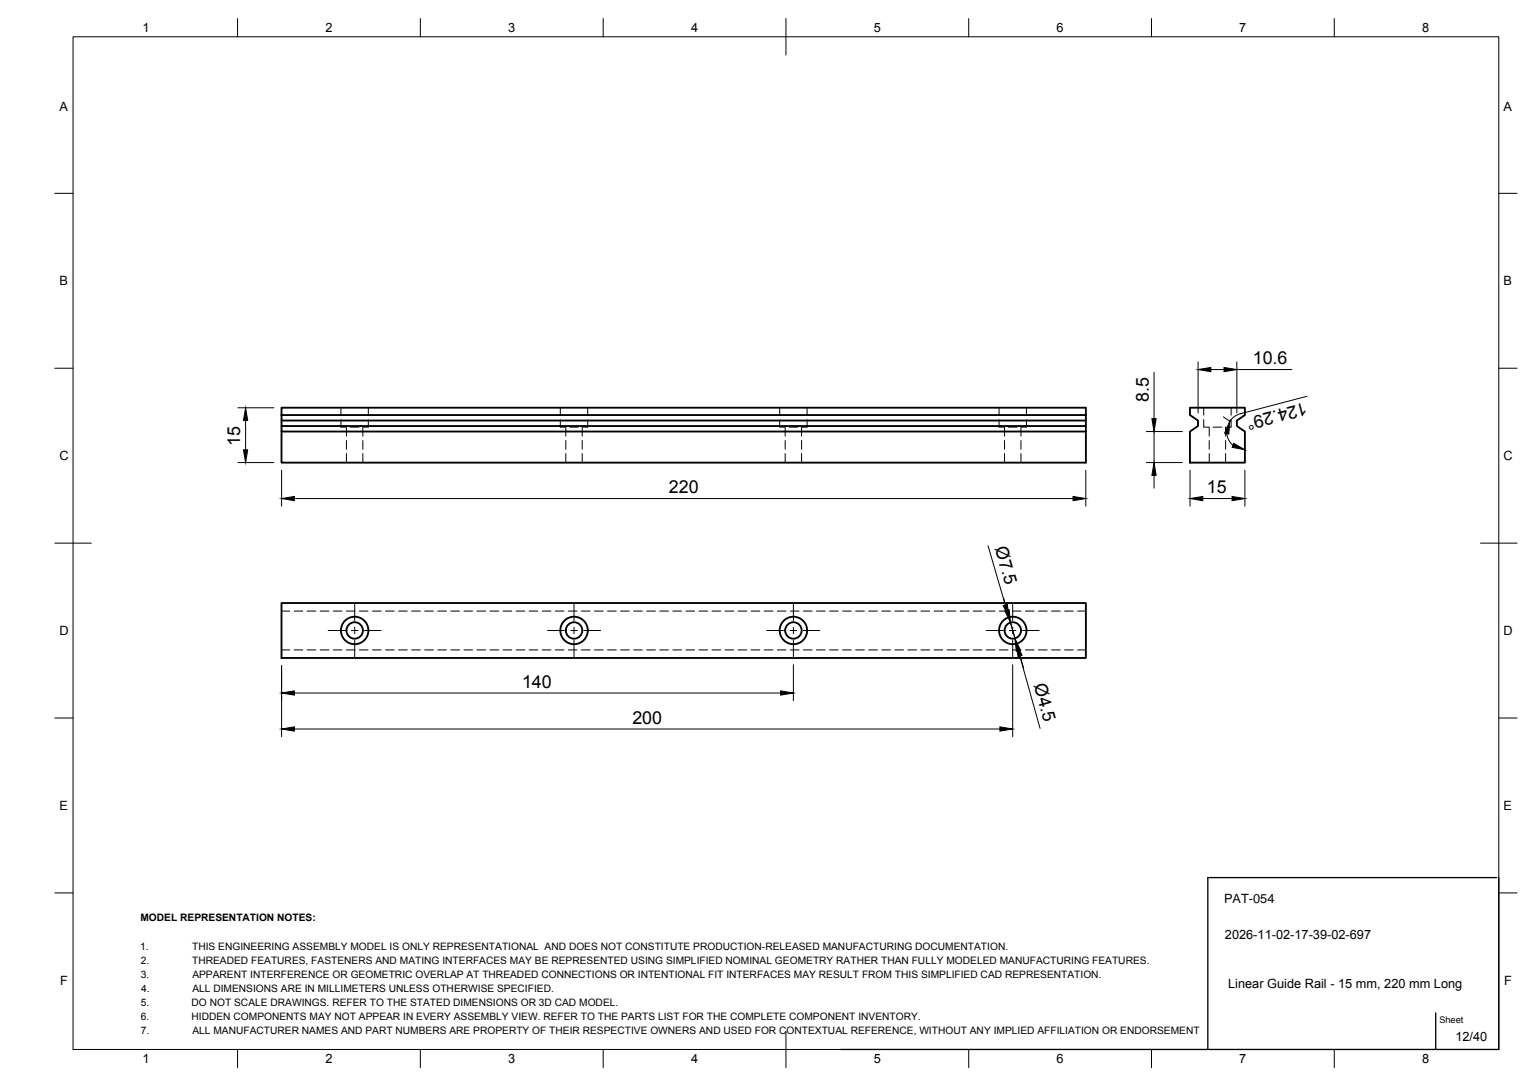
ISO-10303-21;
HEADER;
/* Generated by software containing ST-Developer
 * from STEP Tools, Inc. (www.steptools.com) 
 */

FILE_DESCRIPTION(
/* description */ ('PAT-054'),
/* implementation_level */ '2;1');

FILE_NAME(
/* name */ 'Linear Guide Rail - 15 mm, 220 mm Long.step',
/* time_stamp */ '2026-10-29T16:38:13-07:00',
/* author */ (''),
/* organization */ (''),
/* preprocessor_version */ 'ST-DEVELOPER v20.2',
/* originating_system */ 'Autodesk Translation Framework v15.17.0.0',
/* authorisation */ '');

FILE_SCHEMA (('AUTOMOTIVE_DESIGN { 1 0 10303 214 3 1 1 }'));
ENDSEC;

DATA;
#10=MECHANICAL_DESIGN_GEOMETRIC_PRESENTATION_REPRESENTATION('',(#907),#33981);
#819=SHAPE_REPRESENTATION_RELATIONSHIP('SRR','None',#34192,#863);
#863=ADVANCED_BREP_SHAPE_REPRESENTATION('',(#966),#33940);
#907=STYLED_ITEM('',(#34510),#966);
#966=MANIFOLD_SOLID_BREP('Body1',#13018);
#1116=FACE_BOUND('',#2531,.T.);
#1117=FACE_BOUND('',#2534,.T.);
#1118=FACE_BOUND('',#2537,.T.);
#1119=FACE_BOUND('',#2540,.T.);
#1120=FACE_BOUND('',#2550,.T.);
#1121=FACE_BOUND('',#2551,.T.);
#1122=FACE_BOUND('',#2552,.T.);
#1123=FACE_BOUND('',#2553,.T.);
#1124=FACE_BOUND('',#2560,.T.);
#1125=FACE_BOUND('',#2561,.T.);
#1126=FACE_BOUND('',#2562,.T.);
#1127=FACE_BOUND('',#2563,.T.);
#1293=PLANE('',#13832);
#1294=PLANE('',#13837);
#1295=PLANE('',#13842);
#1296=PLANE('',#13847);
#1297=PLANE('',#13857);
#1298=PLANE('',#13858);
#1299=PLANE('',#13859);
#1300=PLANE('',#13860);
#1301=PLANE('',#13861);
#1302=PLANE('',#13862);
#1303=PLANE('',#13863);
#1304=PLANE('',#13864);
#1305=PLANE('',#13865);
#1306=PLANE('',#13866);
#1307=PLANE('',#13867);
#1308=PLANE('',#13868);
#1309=PLANE('',#13869);
#1310=PLANE('',#13870);
#1702=FACE_OUTER_BOUND('',#2529,.T.);
#1703=FACE_OUTER_BOUND('',#2530,.T.);
#1704=FACE_OUTER_BOUND('',#2532,.T.);
#1705=FACE_OUTER_BOUND('',#2533,.T.);
#1706=FACE_OUTER_BOUND('',#2535,.T.);
#1707=FACE_OUTER_BOUND('',#2536,.T.);
#1708=FACE_OUTER_BOUND('',#2538,.T.);
#1709=FACE_OUTER_BOUND('',#2539,.T.);
#1710=FACE_OUTER_BOUND('',#2541,.T.);
#1711=FACE_OUTER_BOUND('',#2542,.T.);
#1712=FACE_OUTER_BOUND('',#2543,.T.);
#1713=FACE_OUTER_BOUND('',#2544,.T.);
#1714=FACE_OUTER_BOUND('',#2545,.T.);
#1715=FACE_OUTER_BOUND('',#2546,.T.);
#1716=FACE_OUTER_BOUND('',#2547,.T.);
#1717=FACE_OUTER_BOUND('',#2548,.T.);
#1718=FACE_OUTER_BOUND('',#2549,.T.);
#1719=FACE_OUTER_BOUND('',#2554,.T.);
#1720=FACE_OUTER_BOUND('',#2555,.T.);
#1721=FACE_OUTER_BOUND('',#2556,.T.);
#1722=FACE_OUTER_BOUND('',#2557,.T.);
#1723=FACE_OUTER_BOUND('',#2558,.T.);
#1724=FACE_OUTER_BOUND('',#2559,.T.);
#1725=FACE_OUTER_BOUND('',#2564,.T.);
#1726=FACE_OUTER_BOUND('',#2565,.T.);
#1727=FACE_OUTER_BOUND('',#2566,.T.);
#2529=EDGE_LOOP('',(#9107,#9108,#9109,#9110));
#2530=EDGE_LOOP('',(#9111));
#2531=EDGE_LOOP('',(#9112));
#2532=EDGE_LOOP('',(#9113,#9114,#9115,#9116));
#2533=EDGE_LOOP('',(#9117));
#2534=EDGE_LOOP('',(#9118));
#2535=EDGE_LOOP('',(#9119,#9120,#9121,#9122));
#2536=EDGE_LOOP('',(#9123));
#2537=EDGE_LOOP('',(#9124));
#2538=EDGE_LOOP('',(#9125,#9126,#9127,#9128));
#2539=EDGE_LOOP('',(#9129));
#2540=EDGE_LOOP('',(#9130));
#2541=EDGE_LOOP('',(#9131,#9132,#9133,#9134));
#2542=EDGE_LOOP('',(#9135,#9136,#9137,#9138));
#2543=EDGE_LOOP('',(#9139,#9140,#9141,#9142));
#2544=EDGE_LOOP('',(#9143,#9144,#9145,#9146));
#2545=EDGE_LOOP('',(#9147,#9148,#9149,#9150));
#2546=EDGE_LOOP('',(#9151,#9152,#9153,#9154));
#2547=EDGE_LOOP('',(#9155,#9156,#9157,#9158));
#2548=EDGE_LOOP('',(#9159,#9160,#9161,#9162));
#2549=EDGE_LOOP('',(#9163,#9164,#9165,#9166));
#2550=EDGE_LOOP('',(#9167));
#2551=EDGE_LOOP('',(#9168));
#2552=EDGE_LOOP('',(#9169));
#2553=EDGE_LOOP('',(#9170));
#2554=EDGE_LOOP('',(#9171,#9172,#9173,#9174));
#2555=EDGE_LOOP('',(#9175,#9176,#9177,#9178));
#2556=EDGE_LOOP('',(#9179,#9180,#9181,#9182));
#2557=EDGE_LOOP('',(#9183,#9184,#9185,#9186));
#2558=EDGE_LOOP('',(#9187,#9188,#9189,#9190));
#2559=EDGE_LOOP('',(#9191,#9192,#9193,#9194));
#2560=EDGE_LOOP('',(#9195));
#2561=EDGE_LOOP('',(#9196));
#2562=EDGE_LOOP('',(#9197));
#2563=EDGE_LOOP('',(#9198));
#2564=EDGE_LOOP('',(#9199,#9200,#9201,#9202));
#2565=EDGE_LOOP('',(#9203,#9204,#9205,#9206,#9207,#9208,#9209,#9210,#9211,
#9212,#9213,#9214));
#2566=EDGE_LOOP('',(#9215,#9216,#9217,#9218,#9219,#9220,#9221,#9222,#9223,
#9224,#9225,#9226));
#3414=LINE('',#19143,#4348);
#3415=LINE('',#19152,#4349);
#3416=LINE('',#19161,#4350);
#3417=LINE('',#19170,#4351);
#3418=LINE('',#19178,#4352);
#3419=LINE('',#19182,#4353);
#3420=LINE('',#19186,#4354);
#3421=LINE('',#19190,#4355);
#3422=LINE('',#19194,#4356);
#3423=LINE('',#19196,#4357);
#3424=LINE('',#19198,#4358);
#3425=LINE('',#19199,#4359);
#3426=LINE('',#19202,#4360);
#3427=LINE('',#19204,#4361);
#3428=LINE('',#19205,#4362);
#3429=LINE('',#19208,#4363);
#3430=LINE('',#19210,#4364);
#3431=LINE('',#19211,#4365);
#3432=LINE('',#19214,#4366);
#3433=LINE('',#19216,#4367);
#3434=LINE('',#19217,#4368);
#3435=LINE('',#19220,#4369);
#3436=LINE('',#19222,#4370);
#3437=LINE('',#19223,#4371);
#3438=LINE('',#19226,#4372);
#3439=LINE('',#19228,#4373);
#3440=LINE('',#19229,#4374);
#3441=LINE('',#19232,#4375);
#3442=LINE('',#19234,#4376);
#3443=LINE('',#19235,#4377);
#3444=LINE('',#19238,#4378);
#3445=LINE('',#19240,#4379);
#3446=LINE('',#19241,#4380);
#3447=LINE('',#19244,#4381);
#3448=LINE('',#19246,#4382);
#3449=LINE('',#19247,#4383);
#3450=LINE('',#19250,#4384);
#3451=LINE('',#19252,#4385);
#3452=LINE('',#19253,#4386);
#3453=LINE('',#19256,#4387);
#3454=LINE('',#19258,#4388);
#3455=LINE('',#19259,#4389);
#3456=LINE('',#19261,#4390);
#3457=LINE('',#19262,#4391);
#4348=VECTOR('',#15611,0.375);
#4349=VECTOR('',#15622,0.375);
#4350=VECTOR('',#15633,0.375);
#4351=VECTOR('',#15644,0.375);
#4352=VECTOR('',#15655,0.225);
#4353=VECTOR('',#15660,0.225);
#4354=VECTOR('',#15665,0.225);
#4355=VECTOR('',#15670,0.225000000000001);
#4356=VECTOR('',#15673,1.);
#4357=VECTOR('',#15674,1.);
#4358=VECTOR('',#15675,1.);
#4359=VECTOR('',#15676,1.);
#4360=VECTOR('',#15679,1.);
#4361=VECTOR('',#15680,1.);
#4362=VECTOR('',#15681,1.);
#4363=VECTOR('',#15684,1.);
#4364=VECTOR('',#15685,1.);
#4365=VECTOR('',#15686,1.);
#4366=VECTOR('',#15689,1.);
#4367=VECTOR('',#15690,1.);
#4368=VECTOR('',#15691,1.);
#4369=VECTOR('',#15694,1.);
#4370=VECTOR('',#15695,1.);
#4371=VECTOR('',#15696,1.);
#4372=VECTOR('',#15699,1.);
#4373=VECTOR('',#15700,1.);
#4374=VECTOR('',#15701,1.);
#4375=VECTOR('',#15704,1.);
#4376=VECTOR('',#15705,1.);
#4377=VECTOR('',#15706,1.);
#4378=VECTOR('',#15709,1.);
#4379=VECTOR('',#15710,1.);
#4380=VECTOR('',#15711,1.);
#4381=VECTOR('',#15714,1.);
#4382=VECTOR('',#15715,1.);
#4383=VECTOR('',#15716,1.);
#4384=VECTOR('',#15719,1.);
#4385=VECTOR('',#15720,1.);
#4386=VECTOR('',#15721,1.);
#4387=VECTOR('',#15724,1.);
#4388=VECTOR('',#15725,1.);
#4389=VECTOR('',#15726,1.);
#4390=VECTOR('',#15729,1.);
#4391=VECTOR('',#15730,1.);
#5237=CIRCLE('',#13830,0.375);
#5238=CIRCLE('',#13831,0.375);
#5239=CIRCLE('',#13833,0.225);
#5240=CIRCLE('',#13835,0.375);
#5241=CIRCLE('',#13836,0.375);
#5242=CIRCLE('',#13838,0.225);
#5243=CIRCLE('',#13840,0.375);
#5244=CIRCLE('',#13841,0.375);
#5245=CIRCLE('',#13843,0.225);
#5246=CIRCLE('',#13845,0.375);
#5247=CIRCLE('',#13846,0.375);
#5248=CIRCLE('',#13848,0.225000000000001);
#5249=CIRCLE('',#13850,0.225);
#5250=CIRCLE('',#13852,0.225);
#5251=CIRCLE('',#13854,0.225);
#5252=CIRCLE('',#13856,0.225000000000001);
#5776=VERTEX_POINT('',#19140);
#5777=VERTEX_POINT('',#19142);
#5778=VERTEX_POINT('',#19146);
#5779=VERTEX_POINT('',#19149);
#5780=VERTEX_POINT('',#19151);
#5781=VERTEX_POINT('',#19155);
#5782=VERTEX_POINT('',#19158);
#5783=VERTEX_POINT('',#19160);
#5784=VERTEX_POINT('',#19164);
#5785=VERTEX_POINT('',#19167);
#5786=VERTEX_POINT('',#19169);
#5787=VERTEX_POINT('',#19173);
#5788=VERTEX_POINT('',#19176);
#5789=VERTEX_POINT('',#19180);
#5790=VERTEX_POINT('',#19184);
#5791=VERTEX_POINT('',#19188);
#5792=VERTEX_POINT('',#19192);
#5793=VERTEX_POINT('',#19193);
#5794=VERTEX_POINT('',#19195);
#5795=VERTEX_POINT('',#19197);
#5796=VERTEX_POINT('',#19201);
#5797=VERTEX_POINT('',#19203);
#5798=VERTEX_POINT('',#19207);
#5799=VERTEX_POINT('',#19209);
#5800=VERTEX_POINT('',#19213);
#5801=VERTEX_POINT('',#19215);
#5802=VERTEX_POINT('',#19219);
#5803=VERTEX_POINT('',#19221);
#5804=VERTEX_POINT('',#19225);
#5805=VERTEX_POINT('',#19227);
#5806=VERTEX_POINT('',#19231);
#5807=VERTEX_POINT('',#19233);
#5808=VERTEX_POINT('',#19237);
#5809=VERTEX_POINT('',#19239);
#5810=VERTEX_POINT('',#19243);
#5811=VERTEX_POINT('',#19245);
#5812=VERTEX_POINT('',#19249);
#5813=VERTEX_POINT('',#19251);
#5814=VERTEX_POINT('',#19255);
#5815=VERTEX_POINT('',#19257);
#7053=EDGE_CURVE('',#5776,#5776,#5237,.T.);
#7054=EDGE_CURVE('',#5776,#5777,#3414,.T.);
#7055=EDGE_CURVE('',#5777,#5777,#5238,.T.);
#7056=EDGE_CURVE('',#5778,#5778,#5239,.T.);
#7057=EDGE_CURVE('',#5779,#5779,#5240,.T.);
#7058=EDGE_CURVE('',#5779,#5780,#3415,.T.);
#7059=EDGE_CURVE('',#5780,#5780,#5241,.T.);
#7060=EDGE_CURVE('',#5781,#5781,#5242,.T.);
#7061=EDGE_CURVE('',#5782,#5782,#5243,.T.);
#7062=EDGE_CURVE('',#5782,#5783,#3416,.T.);
#7063=EDGE_CURVE('',#5783,#5783,#5244,.T.);
#7064=EDGE_CURVE('',#5784,#5784,#5245,.T.);
#7065=EDGE_CURVE('',#5785,#5785,#5246,.T.);
#7066=EDGE_CURVE('',#5785,#5786,#3417,.T.);
#7067=EDGE_CURVE('',#5786,#5786,#5247,.T.);
#7068=EDGE_CURVE('',#5787,#5787,#5248,.T.);
#7069=EDGE_CURVE('',#5788,#5788,#5249,.T.);
#7070=EDGE_CURVE('',#5788,#5778,#3418,.T.);
#7071=EDGE_CURVE('',#5789,#5789,#5250,.T.);
#7072=EDGE_CURVE('',#5789,#5781,#3419,.T.);
#7073=EDGE_CURVE('',#5790,#5790,#5251,.T.);
#7074=EDGE_CURVE('',#5790,#5784,#3420,.T.);
#7075=EDGE_CURVE('',#5791,#5791,#5252,.T.);
#7076=EDGE_CURVE('',#5791,#5787,#3421,.T.);
#7077=EDGE_CURVE('',#5792,#5793,#3422,.T.);
#7078=EDGE_CURVE('',#5793,#5794,#3423,.T.);
#7079=EDGE_CURVE('',#5795,#5794,#3424,.T.);
#7080=EDGE_CURVE('',#5792,#5795,#3425,.T.);
#7081=EDGE_CURVE('',#5796,#5792,#3426,.T.);
#7082=EDGE_CURVE('',#5797,#5795,#3427,.T.);
#7083=EDGE_CURVE('',#5796,#5797,#3428,.T.);
#7084=EDGE_CURVE('',#5798,#5796,#3429,.T.);
#7085=EDGE_CURVE('',#5799,#5797,#3430,.T.);
#7086=EDGE_CURVE('',#5798,#5799,#3431,.T.);
#7087=EDGE_CURVE('',#5800,#5798,#3432,.T.);
#7088=EDGE_CURVE('',#5801,#5799,#3433,.T.);
#7089=EDGE_CURVE('',#5800,#5801,#3434,.T.);
#7090=EDGE_CURVE('',#5802,#5800,#3435,.T.);
#7091=EDGE_CURVE('',#5803,#5801,#3436,.T.);
#7092=EDGE_CURVE('',#5802,#5803,#3437,.T.);
#7093=EDGE_CURVE('',#5804,#5802,#3438,.T.);
#7094=EDGE_CURVE('',#5805,#5803,#3439,.T.);
#7095=EDGE_CURVE('',#5804,#5805,#3440,.T.);
#7096=EDGE_CURVE('',#5806,#5804,#3441,.T.);
#7097=EDGE_CURVE('',#5807,#5805,#3442,.T.);
#7098=EDGE_CURVE('',#5806,#5807,#3443,.T.);
#7099=EDGE_CURVE('',#5808,#5806,#3444,.T.);
#7100=EDGE_CURVE('',#5809,#5807,#3445,.T.);
#7101=EDGE_CURVE('',#5808,#5809,#3446,.T.);
#7102=EDGE_CURVE('',#5810,#5808,#3447,.T.);
#7103=EDGE_CURVE('',#5811,#5809,#3448,.T.);
#7104=EDGE_CURVE('',#5810,#5811,#3449,.T.);
#7105=EDGE_CURVE('',#5812,#5810,#3450,.T.);
#7106=EDGE_CURVE('',#5813,#5811,#3451,.T.);
#7107=EDGE_CURVE('',#5812,#5813,#3452,.T.);
#7108=EDGE_CURVE('',#5814,#5812,#3453,.T.);
#7109=EDGE_CURVE('',#5815,#5813,#3454,.T.);
#7110=EDGE_CURVE('',#5814,#5815,#3455,.T.);
#7111=EDGE_CURVE('',#5793,#5814,#3456,.T.);
#7112=EDGE_CURVE('',#5794,#5815,#3457,.T.);
#9107=ORIENTED_EDGE('',*,*,#7053,.F.);
#9108=ORIENTED_EDGE('',*,*,#7054,.T.);
#9109=ORIENTED_EDGE('',*,*,#7055,.F.);
#9110=ORIENTED_EDGE('',*,*,#7054,.F.);
#9111=ORIENTED_EDGE('',*,*,#7053,.T.);
#9112=ORIENTED_EDGE('',*,*,#7056,.F.);
#9113=ORIENTED_EDGE('',*,*,#7057,.F.);
#9114=ORIENTED_EDGE('',*,*,#7058,.T.);
#9115=ORIENTED_EDGE('',*,*,#7059,.F.);
#9116=ORIENTED_EDGE('',*,*,#7058,.F.);
#9117=ORIENTED_EDGE('',*,*,#7057,.T.);
#9118=ORIENTED_EDGE('',*,*,#7060,.F.);
#9119=ORIENTED_EDGE('',*,*,#7061,.F.);
#9120=ORIENTED_EDGE('',*,*,#7062,.T.);
#9121=ORIENTED_EDGE('',*,*,#7063,.F.);
#9122=ORIENTED_EDGE('',*,*,#7062,.F.);
#9123=ORIENTED_EDGE('',*,*,#7061,.T.);
#9124=ORIENTED_EDGE('',*,*,#7064,.F.);
#9125=ORIENTED_EDGE('',*,*,#7065,.F.);
#9126=ORIENTED_EDGE('',*,*,#7066,.T.);
#9127=ORIENTED_EDGE('',*,*,#7067,.F.);
#9128=ORIENTED_EDGE('',*,*,#7066,.F.);
#9129=ORIENTED_EDGE('',*,*,#7065,.T.);
#9130=ORIENTED_EDGE('',*,*,#7068,.F.);
#9131=ORIENTED_EDGE('',*,*,#7069,.F.);
#9132=ORIENTED_EDGE('',*,*,#7070,.T.);
#9133=ORIENTED_EDGE('',*,*,#7056,.T.);
#9134=ORIENTED_EDGE('',*,*,#7070,.F.);
#9135=ORIENTED_EDGE('',*,*,#7071,.F.);
#9136=ORIENTED_EDGE('',*,*,#7072,.T.);
#9137=ORIENTED_EDGE('',*,*,#7060,.T.);
#9138=ORIENTED_EDGE('',*,*,#7072,.F.);
#9139=ORIENTED_EDGE('',*,*,#7073,.F.);
#9140=ORIENTED_EDGE('',*,*,#7074,.T.);
#9141=ORIENTED_EDGE('',*,*,#7064,.T.);
#9142=ORIENTED_EDGE('',*,*,#7074,.F.);
#9143=ORIENTED_EDGE('',*,*,#7075,.F.);
#9144=ORIENTED_EDGE('',*,*,#7076,.T.);
#9145=ORIENTED_EDGE('',*,*,#7068,.T.);
#9146=ORIENTED_EDGE('',*,*,#7076,.F.);
#9147=ORIENTED_EDGE('',*,*,#7077,.T.);
#9148=ORIENTED_EDGE('',*,*,#7078,.T.);
#9149=ORIENTED_EDGE('',*,*,#7079,.F.);
#9150=ORIENTED_EDGE('',*,*,#7080,.F.);
#9151=ORIENTED_EDGE('',*,*,#7081,.T.);
#9152=ORIENTED_EDGE('',*,*,#7080,.T.);
#9153=ORIENTED_EDGE('',*,*,#7082,.F.);
#9154=ORIENTED_EDGE('',*,*,#7083,.F.);
#9155=ORIENTED_EDGE('',*,*,#7084,.T.);
#9156=ORIENTED_EDGE('',*,*,#7083,.T.);
#9157=ORIENTED_EDGE('',*,*,#7085,.F.);
#9158=ORIENTED_EDGE('',*,*,#7086,.F.);
#9159=ORIENTED_EDGE('',*,*,#7087,.T.);
#9160=ORIENTED_EDGE('',*,*,#7086,.T.);
#9161=ORIENTED_EDGE('',*,*,#7088,.F.);
#9162=ORIENTED_EDGE('',*,*,#7089,.F.);
#9163=ORIENTED_EDGE('',*,*,#7090,.T.);
#9164=ORIENTED_EDGE('',*,*,#7089,.T.);
#9165=ORIENTED_EDGE('',*,*,#7091,.F.);
#9166=ORIENTED_EDGE('',*,*,#7092,.F.);
#9167=ORIENTED_EDGE('',*,*,#7067,.T.);
#9168=ORIENTED_EDGE('',*,*,#7063,.T.);
#9169=ORIENTED_EDGE('',*,*,#7059,.T.);
#9170=ORIENTED_EDGE('',*,*,#7055,.T.);
#9171=ORIENTED_EDGE('',*,*,#7093,.T.);
#9172=ORIENTED_EDGE('',*,*,#7092,.T.);
#9173=ORIENTED_EDGE('',*,*,#7094,.F.);
#9174=ORIENTED_EDGE('',*,*,#7095,.F.);
#9175=ORIENTED_EDGE('',*,*,#7096,.T.);
#9176=ORIENTED_EDGE('',*,*,#7095,.T.);
#9177=ORIENTED_EDGE('',*,*,#7097,.F.);
#9178=ORIENTED_EDGE('',*,*,#7098,.F.);
#9179=ORIENTED_EDGE('',*,*,#7099,.T.);
#9180=ORIENTED_EDGE('',*,*,#7098,.T.);
#9181=ORIENTED_EDGE('',*,*,#7100,.F.);
#9182=ORIENTED_EDGE('',*,*,#7101,.F.);
#9183=ORIENTED_EDGE('',*,*,#7102,.T.);
#9184=ORIENTED_EDGE('',*,*,#7101,.T.);
#9185=ORIENTED_EDGE('',*,*,#7103,.F.);
#9186=ORIENTED_EDGE('',*,*,#7104,.F.);
#9187=ORIENTED_EDGE('',*,*,#7105,.T.);
#9188=ORIENTED_EDGE('',*,*,#7104,.T.);
#9189=ORIENTED_EDGE('',*,*,#7106,.F.);
#9190=ORIENTED_EDGE('',*,*,#7107,.F.);
#9191=ORIENTED_EDGE('',*,*,#7108,.T.);
#9192=ORIENTED_EDGE('',*,*,#7107,.T.);
#9193=ORIENTED_EDGE('',*,*,#7109,.F.);
#9194=ORIENTED_EDGE('',*,*,#7110,.F.);
#9195=ORIENTED_EDGE('',*,*,#7069,.T.);
#9196=ORIENTED_EDGE('',*,*,#7071,.T.);
#9197=ORIENTED_EDGE('',*,*,#7073,.T.);
#9198=ORIENTED_EDGE('',*,*,#7075,.T.);
#9199=ORIENTED_EDGE('',*,*,#7111,.T.);
#9200=ORIENTED_EDGE('',*,*,#7110,.T.);
#9201=ORIENTED_EDGE('',*,*,#7112,.F.);
#9202=ORIENTED_EDGE('',*,*,#7078,.F.);
#9203=ORIENTED_EDGE('',*,*,#7112,.T.);
#9204=ORIENTED_EDGE('',*,*,#7109,.T.);
#9205=ORIENTED_EDGE('',*,*,#7106,.T.);
#9206=ORIENTED_EDGE('',*,*,#7103,.T.);
#9207=ORIENTED_EDGE('',*,*,#7100,.T.);
#9208=ORIENTED_EDGE('',*,*,#7097,.T.);
#9209=ORIENTED_EDGE('',*,*,#7094,.T.);
#9210=ORIENTED_EDGE('',*,*,#7091,.T.);
#9211=ORIENTED_EDGE('',*,*,#7088,.T.);
#9212=ORIENTED_EDGE('',*,*,#7085,.T.);
#9213=ORIENTED_EDGE('',*,*,#7082,.T.);
#9214=ORIENTED_EDGE('',*,*,#7079,.T.);
#9215=ORIENTED_EDGE('',*,*,#7111,.F.);
#9216=ORIENTED_EDGE('',*,*,#7077,.F.);
#9217=ORIENTED_EDGE('',*,*,#7081,.F.);
#9218=ORIENTED_EDGE('',*,*,#7084,.F.);
#9219=ORIENTED_EDGE('',*,*,#7087,.F.);
#9220=ORIENTED_EDGE('',*,*,#7090,.F.);
#9221=ORIENTED_EDGE('',*,*,#7093,.F.);
#9222=ORIENTED_EDGE('',*,*,#7096,.F.);
#9223=ORIENTED_EDGE('',*,*,#7099,.F.);
#9224=ORIENTED_EDGE('',*,*,#7102,.F.);
#9225=ORIENTED_EDGE('',*,*,#7105,.F.);
#9226=ORIENTED_EDGE('',*,*,#7108,.F.);
#12041=CYLINDRICAL_SURFACE('',#13829,0.375);
#12042=CYLINDRICAL_SURFACE('',#13834,0.375);
#12043=CYLINDRICAL_SURFACE('',#13839,0.375);
#12044=CYLINDRICAL_SURFACE('',#13844,0.375);
#12045=CYLINDRICAL_SURFACE('',#13849,0.225);
#12046=CYLINDRICAL_SURFACE('',#13851,0.225);
#12047=CYLINDRICAL_SURFACE('',#13853,0.225);
#12048=CYLINDRICAL_SURFACE('',#13855,0.225000000000001);
#12414=ADVANCED_FACE('',(#1702),#12041,.F.);
#12415=ADVANCED_FACE('',(#1703,#1116),#1293,.T.);
#12416=ADVANCED_FACE('',(#1704),#12042,.F.);
#12417=ADVANCED_FACE('',(#1705,#1117),#1294,.T.);
#12418=ADVANCED_FACE('',(#1706),#12043,.F.);
#12419=ADVANCED_FACE('',(#1707,#1118),#1295,.T.);
#12420=ADVANCED_FACE('',(#1708),#12044,.F.);
#12421=ADVANCED_FACE('',(#1709,#1119),#1296,.T.);
#12422=ADVANCED_FACE('',(#1710),#12045,.F.);
#12423=ADVANCED_FACE('',(#1711),#12046,.F.);
#12424=ADVANCED_FACE('',(#1712),#12047,.F.);
#12425=ADVANCED_FACE('',(#1713),#12048,.F.);
#12426=ADVANCED_FACE('',(#1714),#1297,.T.);
#12427=ADVANCED_FACE('',(#1715),#1298,.T.);
#12428=ADVANCED_FACE('',(#1716),#1299,.T.);
#12429=ADVANCED_FACE('',(#1717),#1300,.T.);
#12430=ADVANCED_FACE('',(#1718,#1120,#1121,#1122,#1123),#1301,.T.);
#12431=ADVANCED_FACE('',(#1719),#1302,.T.);
#12432=ADVANCED_FACE('',(#1720),#1303,.T.);
#12433=ADVANCED_FACE('',(#1721),#1304,.T.);
#12434=ADVANCED_FACE('',(#1722),#1305,.T.);
#12435=ADVANCED_FACE('',(#1723),#1306,.T.);
#12436=ADVANCED_FACE('',(#1724,#1124,#1125,#1126,#1127),#1307,.T.);
#12437=ADVANCED_FACE('',(#1725),#1308,.T.);
#12438=ADVANCED_FACE('',(#1726),#1309,.T.);
#12439=ADVANCED_FACE('',(#1727),#1310,.F.);
#13018=CLOSED_SHELL('',(#12414,#12415,#12416,#12417,#12418,#12419,#12420,
#12421,#12422,#12423,#12424,#12425,#12426,#12427,#12428,#12429,#12430,#12431,
#12432,#12433,#12434,#12435,#12436,#12437,#12438,#12439));
#13828=AXIS2_PLACEMENT_3D('',#19138,#15605,#15606);
#13829=AXIS2_PLACEMENT_3D('',#19139,#15607,#15608);
#13830=AXIS2_PLACEMENT_3D('',#19141,#15609,#15610);
#13831=AXIS2_PLACEMENT_3D('',#19144,#15612,#15613);
#13832=AXIS2_PLACEMENT_3D('',#19145,#15614,#15615);
#13833=AXIS2_PLACEMENT_3D('',#19147,#15616,#15617);
#13834=AXIS2_PLACEMENT_3D('',#19148,#15618,#15619);
#13835=AXIS2_PLACEMENT_3D('',#19150,#15620,#15621);
#13836=AXIS2_PLACEMENT_3D('',#19153,#15623,#15624);
#13837=AXIS2_PLACEMENT_3D('',#19154,#15625,#15626);
#13838=AXIS2_PLACEMENT_3D('',#19156,#15627,#15628);
#13839=AXIS2_PLACEMENT_3D('',#19157,#15629,#15630);
#13840=AXIS2_PLACEMENT_3D('',#19159,#15631,#15632);
#13841=AXIS2_PLACEMENT_3D('',#19162,#15634,#15635);
#13842=AXIS2_PLACEMENT_3D('',#19163,#15636,#15637);
#13843=AXIS2_PLACEMENT_3D('',#19165,#15638,#15639);
#13844=AXIS2_PLACEMENT_3D('',#19166,#15640,#15641);
#13845=AXIS2_PLACEMENT_3D('',#19168,#15642,#15643);
#13846=AXIS2_PLACEMENT_3D('',#19171,#15645,#15646);
#13847=AXIS2_PLACEMENT_3D('',#19172,#15647,#15648);
#13848=AXIS2_PLACEMENT_3D('',#19174,#15649,#15650);
#13849=AXIS2_PLACEMENT_3D('',#19175,#15651,#15652);
#13850=AXIS2_PLACEMENT_3D('',#19177,#15653,#15654);
#13851=AXIS2_PLACEMENT_3D('',#19179,#15656,#15657);
#13852=AXIS2_PLACEMENT_3D('',#19181,#15658,#15659);
#13853=AXIS2_PLACEMENT_3D('',#19183,#15661,#15662);
#13854=AXIS2_PLACEMENT_3D('',#19185,#15663,#15664);
#13855=AXIS2_PLACEMENT_3D('',#19187,#15666,#15667);
#13856=AXIS2_PLACEMENT_3D('',#19189,#15668,#15669);
#13857=AXIS2_PLACEMENT_3D('',#19191,#15671,#15672);
#13858=AXIS2_PLACEMENT_3D('',#19200,#15677,#15678);
#13859=AXIS2_PLACEMENT_3D('',#19206,#15682,#15683);
#13860=AXIS2_PLACEMENT_3D('',#19212,#15687,#15688);
#13861=AXIS2_PLACEMENT_3D('',#19218,#15692,#15693);
#13862=AXIS2_PLACEMENT_3D('',#19224,#15697,#15698);
#13863=AXIS2_PLACEMENT_3D('',#19230,#15702,#15703);
#13864=AXIS2_PLACEMENT_3D('',#19236,#15707,#15708);
#13865=AXIS2_PLACEMENT_3D('',#19242,#15712,#15713);
#13866=AXIS2_PLACEMENT_3D('',#19248,#15717,#15718);
#13867=AXIS2_PLACEMENT_3D('',#19254,#15722,#15723);
#13868=AXIS2_PLACEMENT_3D('',#19260,#15727,#15728);
#13869=AXIS2_PLACEMENT_3D('',#19263,#15731,#15732);
#13870=AXIS2_PLACEMENT_3D('',#19264,#15733,#15734);
#15605=DIRECTION('axis',(0.,0.,1.));
#15606=DIRECTION('refdir',(1.,0.,0.));
#15607=DIRECTION('center_axis',(0.,0.,1.));
#15608=DIRECTION('ref_axis',(1.,0.,0.));
#15609=DIRECTION('center_axis',(0.,0.,1.));
#15610=DIRECTION('ref_axis',(1.,0.,0.));
#15611=DIRECTION('',(0.,0.,1.));
#15612=DIRECTION('center_axis',(0.,0.,-1.));
#15613=DIRECTION('ref_axis',(1.,0.,0.));
#15614=DIRECTION('center_axis',(0.,0.,1.));
#15615=DIRECTION('ref_axis',(1.,0.,0.));
#15616=DIRECTION('center_axis',(0.,0.,1.));
#15617=DIRECTION('ref_axis',(1.,0.,0.));
#15618=DIRECTION('center_axis',(0.,0.,1.));
#15619=DIRECTION('ref_axis',(1.,0.,0.));
#15620=DIRECTION('center_axis',(0.,0.,1.));
#15621=DIRECTION('ref_axis',(1.,0.,0.));
#15622=DIRECTION('',(0.,0.,1.));
#15623=DIRECTION('center_axis',(0.,0.,-1.));
#15624=DIRECTION('ref_axis',(1.,0.,0.));
#15625=DIRECTION('center_axis',(0.,0.,1.));
#15626=DIRECTION('ref_axis',(1.,0.,0.));
#15627=DIRECTION('center_axis',(0.,0.,1.));
#15628=DIRECTION('ref_axis',(1.,0.,0.));
#15629=DIRECTION('center_axis',(0.,0.,1.));
#15630=DIRECTION('ref_axis',(1.,0.,0.));
#15631=DIRECTION('center_axis',(0.,0.,1.));
#15632=DIRECTION('ref_axis',(1.,0.,0.));
#15633=DIRECTION('',(0.,0.,1.));
#15634=DIRECTION('center_axis',(0.,0.,-1.));
#15635=DIRECTION('ref_axis',(1.,0.,0.));
#15636=DIRECTION('center_axis',(0.,0.,1.));
#15637=DIRECTION('ref_axis',(1.,0.,0.));
#15638=DIRECTION('center_axis',(0.,0.,1.));
#15639=DIRECTION('ref_axis',(1.,0.,0.));
#15640=DIRECTION('center_axis',(0.,0.,1.));
#15641=DIRECTION('ref_axis',(1.,0.,0.));
#15642=DIRECTION('center_axis',(0.,0.,1.));
#15643=DIRECTION('ref_axis',(1.,0.,0.));
#15644=DIRECTION('',(0.,0.,1.));
#15645=DIRECTION('center_axis',(0.,0.,-1.));
#15646=DIRECTION('ref_axis',(1.,0.,0.));
#15647=DIRECTION('center_axis',(0.,0.,1.));
#15648=DIRECTION('ref_axis',(1.,0.,0.));
#15649=DIRECTION('center_axis',(0.,0.,1.));
#15650=DIRECTION('ref_axis',(1.,0.,0.));
#15651=DIRECTION('center_axis',(0.,0.,1.));
#15652=DIRECTION('ref_axis',(1.,0.,0.));
#15653=DIRECTION('center_axis',(0.,0.,1.));
#15654=DIRECTION('ref_axis',(1.,0.,0.));
#15655=DIRECTION('',(0.,0.,1.));
#15656=DIRECTION('center_axis',(0.,0.,1.));
#15657=DIRECTION('ref_axis',(1.,0.,0.));
#15658=DIRECTION('center_axis',(0.,0.,1.));
#15659=DIRECTION('ref_axis',(1.,0.,0.));
#15660=DIRECTION('',(0.,0.,1.));
#15661=DIRECTION('center_axis',(0.,0.,1.));
#15662=DIRECTION('ref_axis',(1.,0.,0.));
#15663=DIRECTION('center_axis',(0.,0.,1.));
#15664=DIRECTION('ref_axis',(1.,0.,0.));
#15665=DIRECTION('',(0.,0.,1.));
#15666=DIRECTION('center_axis',(0.,0.,1.));
#15667=DIRECTION('ref_axis',(1.,0.,0.));
#15668=DIRECTION('center_axis',(0.,0.,1.));
#15669=DIRECTION('ref_axis',(1.,0.,0.));
#15670=DIRECTION('',(0.,0.,1.));
#15671=DIRECTION('center_axis',(0.,-0.56333682464151,0.826227342807548));
#15672=DIRECTION('ref_axis',(0.,-0.826227342807548,-0.56333682464151));
#15673=DIRECTION('',(0.,-0.826227342807548,-0.56333682464151));
#15674=DIRECTION('',(1.,0.,0.));
#15675=DIRECTION('',(0.,-0.826227342807548,-0.56333682464151));
#15676=DIRECTION('',(1.,0.,0.));
#15677=DIRECTION('center_axis',(0.,-1.,0.));
#15678=DIRECTION('ref_axis',(0.,0.,-1.));
#15679=DIRECTION('',(0.,0.,-1.));
#15680=DIRECTION('',(0.,0.,-1.));
#15681=DIRECTION('',(1.,0.,0.));
#15682=DIRECTION('center_axis',(0.,-0.56333682464151,-0.826227342807548));
#15683=DIRECTION('ref_axis',(0.,0.826227342807548,-0.56333682464151));
#15684=DIRECTION('',(0.,0.826227342807548,-0.56333682464151));
#15685=DIRECTION('',(0.,0.826227342807548,-0.56333682464151));
#15686=DIRECTION('',(1.,0.,0.));
#15687=DIRECTION('center_axis',(0.,-1.,0.));
#15688=DIRECTION('ref_axis',(0.,0.,-1.));
#15689=DIRECTION('',(0.,0.,-1.));
#15690=DIRECTION('',(0.,0.,-1.));
#15691=DIRECTION('',(1.,0.,0.));
#15692=DIRECTION('center_axis',(0.,0.,1.));
#15693=DIRECTION('ref_axis',(0.,-1.,0.));
#15694=DIRECTION('',(0.,-1.,0.));
#15695=DIRECTION('',(0.,-1.,0.));
#15696=DIRECTION('',(1.,0.,0.));
#15697=DIRECTION('center_axis',(0.,1.,0.));
#15698=DIRECTION('ref_axis',(0.,0.,1.));
#15699=DIRECTION('',(0.,0.,1.));
#15700=DIRECTION('',(0.,0.,1.));
#15701=DIRECTION('',(1.,0.,0.));
#15702=DIRECTION('center_axis',(0.,0.56333682464151,-0.826227342807548));
#15703=DIRECTION('ref_axis',(0.,0.826227342807548,0.56333682464151));
#15704=DIRECTION('',(0.,0.826227342807548,0.56333682464151));
#15705=DIRECTION('',(0.,0.826227342807548,0.56333682464151));
#15706=DIRECTION('',(1.,0.,0.));
#15707=DIRECTION('center_axis',(0.,1.,0.));
#15708=DIRECTION('ref_axis',(0.,0.,1.));
#15709=DIRECTION('',(0.,0.,1.));
#15710=DIRECTION('',(0.,0.,1.));
#15711=DIRECTION('',(1.,0.,0.));
#15712=DIRECTION('center_axis',(0.,0.56333682464151,0.826227342807548));
#15713=DIRECTION('ref_axis',(0.,-0.826227342807548,0.56333682464151));
#15714=DIRECTION('',(0.,-0.826227342807548,0.56333682464151));
#15715=DIRECTION('',(0.,-0.826227342807548,0.56333682464151));
#15716=DIRECTION('',(1.,0.,0.));
#15717=DIRECTION('center_axis',(0.,1.,0.));
#15718=DIRECTION('ref_axis',(0.,0.,1.));
#15719=DIRECTION('',(0.,0.,1.));
#15720=DIRECTION('',(0.,0.,1.));
#15721=DIRECTION('',(1.,0.,0.));
#15722=DIRECTION('center_axis',(0.,0.,-1.));
#15723=DIRECTION('ref_axis',(0.,1.,0.));
#15724=DIRECTION('',(0.,1.,0.));
#15725=DIRECTION('',(0.,1.,0.));
#15726=DIRECTION('',(1.,0.,0.));
#15727=DIRECTION('center_axis',(0.,-1.,0.));
#15728=DIRECTION('ref_axis',(0.,0.,-1.));
#15729=DIRECTION('',(0.,0.,-1.));
#15730=DIRECTION('',(0.,0.,-1.));
#15731=DIRECTION('center_axis',(1.,0.,0.));
#15732=DIRECTION('ref_axis',(0.,0.,-1.));
#15733=DIRECTION('center_axis',(1.,0.,0.));
#15734=DIRECTION('ref_axis',(0.,0.,-1.));
#19138=CARTESIAN_POINT('',(0.,0.,0.));
#19139=CARTESIAN_POINT('Origin',(14.,0.,0.97));
#19140=CARTESIAN_POINT('',(13.625,-4.59242549680257E-17,0.97));
#19141=CARTESIAN_POINT('Origin',(14.,0.,0.97));
#19142=CARTESIAN_POINT('',(13.625,4.59242549680257E-17,1.5));
#19143=CARTESIAN_POINT('',(13.625,-4.59242549680257E-17,0.97));
#19144=CARTESIAN_POINT('Origin',(14.,0.,1.5));
#19145=CARTESIAN_POINT('Origin',(14.,0.,0.97));
#19146=CARTESIAN_POINT('',(13.775,-2.75545529808154E-17,0.97));
#19147=CARTESIAN_POINT('Origin',(14.,0.,0.97));
#19148=CARTESIAN_POINT('Origin',(8.,0.,0.97));
#19149=CARTESIAN_POINT('',(7.625,-4.59242549680257E-17,0.97));
#19150=CARTESIAN_POINT('Origin',(8.,0.,0.97));
#19151=CARTESIAN_POINT('',(7.625,4.59242549680257E-17,1.5));
#19152=CARTESIAN_POINT('',(7.625,-4.59242549680257E-17,0.97));
#19153=CARTESIAN_POINT('Origin',(8.,0.,1.5));
#19154=CARTESIAN_POINT('Origin',(8.,0.,0.97));
#19155=CARTESIAN_POINT('',(7.775,-2.75545529808154E-17,0.97));
#19156=CARTESIAN_POINT('Origin',(8.,0.,0.97));
#19157=CARTESIAN_POINT('Origin',(2.,0.,0.97));
#19158=CARTESIAN_POINT('',(1.625,-4.59242549680257E-17,0.97));
#19159=CARTESIAN_POINT('Origin',(2.,0.,0.97));
#19160=CARTESIAN_POINT('',(1.625,4.59242549680257E-17,1.5));
#19161=CARTESIAN_POINT('',(1.625,-4.59242549680257E-17,0.97));
#19162=CARTESIAN_POINT('Origin',(2.,0.,1.5));
#19163=CARTESIAN_POINT('Origin',(2.,0.,0.97));
#19164=CARTESIAN_POINT('',(1.775,-2.75545529808155E-17,0.97));
#19165=CARTESIAN_POINT('Origin',(2.,0.,0.97));
#19166=CARTESIAN_POINT('Origin',(20.,0.,0.97));
#19167=CARTESIAN_POINT('',(19.625,-4.59242549680257E-17,0.97));
#19168=CARTESIAN_POINT('Origin',(20.,0.,0.97));
#19169=CARTESIAN_POINT('',(19.625,4.59242549680257E-17,1.5));
#19170=CARTESIAN_POINT('',(19.625,-4.59242549680257E-17,0.97));
#19171=CARTESIAN_POINT('Origin',(20.,0.,1.5));
#19172=CARTESIAN_POINT('Origin',(20.,0.,0.97));
#19173=CARTESIAN_POINT('',(19.775,-2.75545529808156E-17,0.97));
#19174=CARTESIAN_POINT('Origin',(20.,0.,0.97));
#19175=CARTESIAN_POINT('Origin',(14.,0.,-0.1));
#19176=CARTESIAN_POINT('',(13.775,-2.75545529808154E-17,0.));
#19177=CARTESIAN_POINT('Origin',(14.,0.,0.));
#19178=CARTESIAN_POINT('',(13.775,-2.75545529808154E-17,-0.1));
#19179=CARTESIAN_POINT('Origin',(8.,0.,-0.1));
#19180=CARTESIAN_POINT('',(7.775,-2.75545529808154E-17,0.));
#19181=CARTESIAN_POINT('Origin',(8.,0.,0.));
#19182=CARTESIAN_POINT('',(7.775,-2.75545529808154E-17,-0.1));
#19183=CARTESIAN_POINT('Origin',(2.,0.,-0.1));
#19184=CARTESIAN_POINT('',(1.775,-2.75545529808155E-17,0.));
#19185=CARTESIAN_POINT('Origin',(2.,0.,0.));
#19186=CARTESIAN_POINT('',(1.775,-2.75545529808155E-17,-0.1));
#19187=CARTESIAN_POINT('Origin',(20.,0.,-0.1));
#19188=CARTESIAN_POINT('',(19.775,-2.75545529808156E-17,0.));
#19189=CARTESIAN_POINT('Origin',(20.,0.,0.));
#19190=CARTESIAN_POINT('',(19.775,-2.75545529808156E-17,-0.1));
#19191=CARTESIAN_POINT('Origin',(0.,-0.53,1.));
#19192=CARTESIAN_POINT('',(0.,-0.53,1.));
#19193=CARTESIAN_POINT('',(0.,-0.75,0.85));
#19194=CARTESIAN_POINT('',(0.,-0.53,1.));
#19195=CARTESIAN_POINT('',(22.,-0.75,0.85));
#19196=CARTESIAN_POINT('',(0.,-0.75,0.85));
#19197=CARTESIAN_POINT('',(22.,-0.53,1.));
#19198=CARTESIAN_POINT('',(22.,-0.53,1.));
#19199=CARTESIAN_POINT('',(0.,-0.53,1.));
#19200=CARTESIAN_POINT('Origin',(0.,-0.53,1.15));
#19201=CARTESIAN_POINT('',(0.,-0.53,1.15));
#19202=CARTESIAN_POINT('',(0.,-0.53,1.15));
#19203=CARTESIAN_POINT('',(22.,-0.53,1.15));
#19204=CARTESIAN_POINT('',(22.,-0.53,1.15));
#19205=CARTESIAN_POINT('',(0.,-0.53,1.15));
#19206=CARTESIAN_POINT('Origin',(0.,-0.75,1.3));
#19207=CARTESIAN_POINT('',(0.,-0.75,1.3));
#19208=CARTESIAN_POINT('',(0.,-0.75,1.3));
#19209=CARTESIAN_POINT('',(22.,-0.75,1.3));
#19210=CARTESIAN_POINT('',(22.,-0.75,1.3));
#19211=CARTESIAN_POINT('',(0.,-0.75,1.3));
#19212=CARTESIAN_POINT('Origin',(0.,-0.75,1.5));
#19213=CARTESIAN_POINT('',(0.,-0.75,1.5));
#19214=CARTESIAN_POINT('',(0.,-0.75,1.5));
#19215=CARTESIAN_POINT('',(22.,-0.75,1.5));
#19216=CARTESIAN_POINT('',(22.,-0.75,1.5));
#19217=CARTESIAN_POINT('',(0.,-0.75,1.5));
#19218=CARTESIAN_POINT('Origin',(0.,0.75,1.5));
#19219=CARTESIAN_POINT('',(0.,0.75,1.5));
#19220=CARTESIAN_POINT('',(0.,0.75,1.5));
#19221=CARTESIAN_POINT('',(22.,0.75,1.5));
#19222=CARTESIAN_POINT('',(22.,0.75,1.5));
#19223=CARTESIAN_POINT('',(0.,0.75,1.5));
#19224=CARTESIAN_POINT('Origin',(0.,0.75,1.3));
#19225=CARTESIAN_POINT('',(0.,0.75,1.3));
#19226=CARTESIAN_POINT('',(0.,0.75,1.3));
#19227=CARTESIAN_POINT('',(22.,0.75,1.3));
#19228=CARTESIAN_POINT('',(22.,0.75,1.3));
#19229=CARTESIAN_POINT('',(0.,0.75,1.3));
#19230=CARTESIAN_POINT('Origin',(0.,0.53,1.15));
#19231=CARTESIAN_POINT('',(0.,0.53,1.15));
#19232=CARTESIAN_POINT('',(0.,0.53,1.15));
#19233=CARTESIAN_POINT('',(22.,0.53,1.15));
#19234=CARTESIAN_POINT('',(22.,0.53,1.15));
#19235=CARTESIAN_POINT('',(0.,0.53,1.15));
#19236=CARTESIAN_POINT('Origin',(0.,0.53,1.));
#19237=CARTESIAN_POINT('',(0.,0.53,1.));
#19238=CARTESIAN_POINT('',(0.,0.53,1.));
#19239=CARTESIAN_POINT('',(22.,0.53,1.));
#19240=CARTESIAN_POINT('',(22.,0.53,1.));
#19241=CARTESIAN_POINT('',(0.,0.53,1.));
#19242=CARTESIAN_POINT('Origin',(0.,0.75,0.85));
#19243=CARTESIAN_POINT('',(0.,0.75,0.85));
#19244=CARTESIAN_POINT('',(0.,0.75,0.85));
#19245=CARTESIAN_POINT('',(22.,0.75,0.85));
#19246=CARTESIAN_POINT('',(22.,0.75,0.85));
#19247=CARTESIAN_POINT('',(0.,0.75,0.85));
#19248=CARTESIAN_POINT('Origin',(0.,0.75,0.));
#19249=CARTESIAN_POINT('',(0.,0.75,0.));
#19250=CARTESIAN_POINT('',(0.,0.75,0.));
#19251=CARTESIAN_POINT('',(22.,0.75,0.));
#19252=CARTESIAN_POINT('',(22.,0.75,0.));
#19253=CARTESIAN_POINT('',(0.,0.75,0.));
#19254=CARTESIAN_POINT('Origin',(0.,-0.75,0.));
#19255=CARTESIAN_POINT('',(0.,-0.75,0.));
#19256=CARTESIAN_POINT('',(0.,-0.75,0.));
#19257=CARTESIAN_POINT('',(22.,-0.75,0.));
#19258=CARTESIAN_POINT('',(22.,-0.75,0.));
#19259=CARTESIAN_POINT('',(0.,-0.75,0.));
#19260=CARTESIAN_POINT('Origin',(0.,-0.75,0.85));
#19261=CARTESIAN_POINT('',(0.,-0.75,0.85));
#19262=CARTESIAN_POINT('',(22.,-0.75,0.85));
#19263=CARTESIAN_POINT('Origin',(22.,0.,0.75));
#19264=CARTESIAN_POINT('Origin',(0.,0.,0.75));
#33888=UNCERTAINTY_MEASURE_WITH_UNIT(LENGTH_MEASURE(0.001),#33982,
'DISTANCE_ACCURACY_VALUE',
'Maximum model space distance between geometric entities at asserted c
onnectivities');
#33929=UNCERTAINTY_MEASURE_WITH_UNIT(LENGTH_MEASURE(0.001),#33982,
'DISTANCE_ACCURACY_VALUE',
'Maximum model space distance between geometric entities at asserted c
onnectivities');
#33940=(
GEOMETRIC_REPRESENTATION_CONTEXT(3)
GLOBAL_UNCERTAINTY_ASSIGNED_CONTEXT((#33888))
GLOBAL_UNIT_ASSIGNED_CONTEXT((#33982,#33984,#33985))
REPRESENTATION_CONTEXT('','3D')
);
#33981=(
GEOMETRIC_REPRESENTATION_CONTEXT(3)
GLOBAL_UNCERTAINTY_ASSIGNED_CONTEXT((#33929))
GLOBAL_UNIT_ASSIGNED_CONTEXT((#33982,#33984,#33985))
REPRESENTATION_CONTEXT('','3D')
);
#33982=(
LENGTH_UNIT()
NAMED_UNIT(*)
SI_UNIT(.CENTI.,.METRE.)
);
#33984=(
NAMED_UNIT(*)
PLANE_ANGLE_UNIT()
SI_UNIT($,.RADIAN.)
);
#33985=(
NAMED_UNIT(*)
SI_UNIT($,.STERADIAN.)
SOLID_ANGLE_UNIT()
);
#33996=SHAPE_DEFINITION_REPRESENTATION(#34047,#34192);
#34047=PRODUCT_DEFINITION_SHAPE('',$,#34244);
#34192=SHAPE_REPRESENTATION('',(#13828),#33940);
#34233=PRODUCT_DEFINITION_CONTEXT('part definition',#34388,'design');
#34244=PRODUCT_DEFINITION('Linear Guide Rail - 15 mm, 220 mm Long',
'Linear Guide Rail - 15 mm, 220 mm Long',#34295,#34233);
#34295=PRODUCT_DEFINITION_FORMATION('',$,#34400);
#34388=APPLICATION_CONTEXT(
'Core Data for Automotive Mechanical Design Process');
#34389=PRODUCT_CONTEXT('part definition',#34388,'mechanical');
#34400=PRODUCT('Linear Guide Rail - 15 mm, 220 mm Long',
'Linear Guide Rail - 15 mm, 220 mm Long',
'Linear Guide Rail - 15 mm, 220 mm Long',(#34389));
#34504=COLOUR_RGB('Sky Blue',0.24,0.69,0.87);
#34505=FILL_AREA_STYLE_COLOUR('',#34504);
#34506=FILL_AREA_STYLE('',(#34505));
#34507=SURFACE_STYLE_FILL_AREA(#34506);
#34508=SURFACE_SIDE_STYLE('',(#34507));
#34509=SURFACE_STYLE_USAGE(.BOTH.,#34508);
#34510=PRESENTATION_STYLE_ASSIGNMENT((#34509));
ENDSEC;
END-ISO-10303-21;
